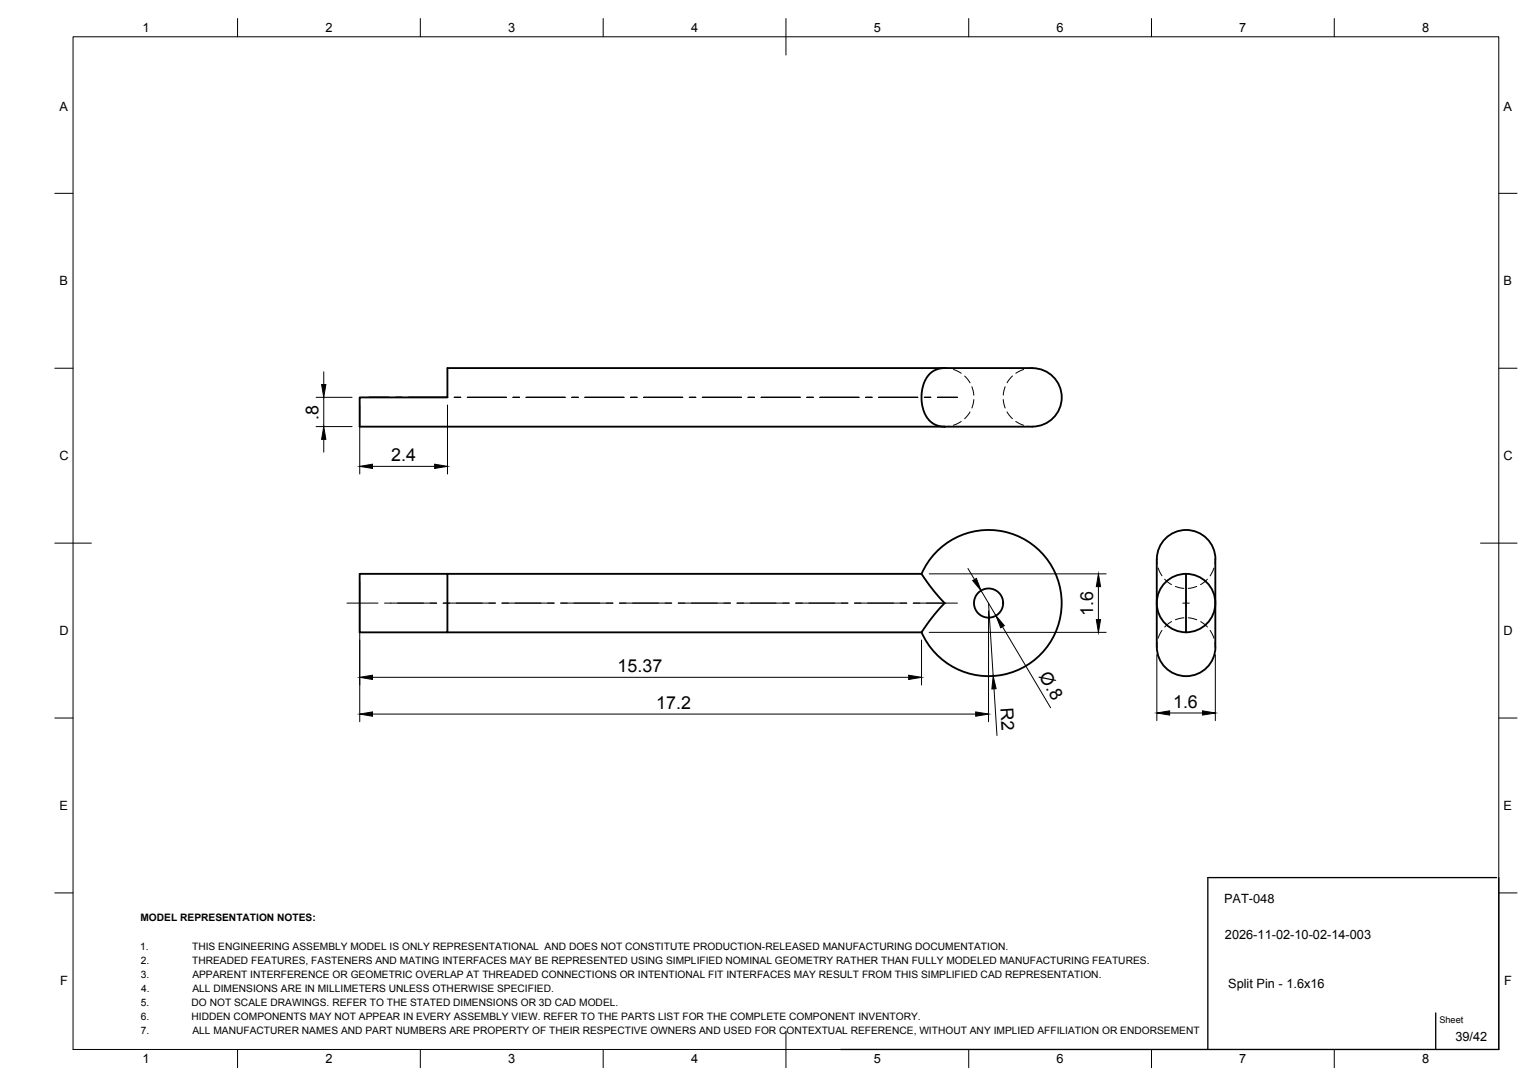
ISO-10303-21;
HEADER;
/* Generated by software containing ST-Developer
 * from STEP Tools, Inc. (www.steptools.com) 
 */

FILE_DESCRIPTION(
/* description */ ('Guided pneumatic stop gate'),
/* implementation_level */ '2;1');

FILE_NAME(
/* name */ 'Split Pin - 1.6x16.step',
/* time_stamp */ '2026-10-27T21:43:45-07:00',
/* author */ (''),
/* organization */ (''),
/* preprocessor_version */ 'ST-DEVELOPER v20.2',
/* originating_system */ 'Autodesk Translation Framework v15.17.0.0',
/* authorisation */ '');

FILE_SCHEMA (('AUTOMOTIVE_DESIGN { 1 0 10303 214 3 1 1 }'));
ENDSEC;

DATA;
#10=MECHANICAL_DESIGN_GEOMETRIC_PRESENTATION_REPRESENTATION('',(#571),#14392);
#17=B_SPLINE_CURVE_WITH_KNOTS('',3,(#14014,#14015,#14016,#14017,#14018,
#14019,#14020,#14021,#14022,#14023,#14024,#14025,#14026,#14027,#14028,#14029,
#14030,#14031,#14032,#14033,#14034,#14035,#14036,#14037,#14038,#14039),
 .UNSPECIFIED.,.F.,.F.,(4,2,2,2,2,2,2,2,2,2,2,2,4),(-0.00054581412719389,
0.,0.0281583564005144,0.0618496465371181,0.0905865724114538,0.120694112793616,
0.144966158459363,0.16923820412511,0.199345744507272,0.228082670381608,
0.261773960518212,0.289932316918681,0.290478131045882),.UNSPECIFIED.);
#18=B_SPLINE_CURVE_WITH_KNOTS('',3,(#14040,#14041,#14042,#14043,#14044,
#14045,#14046,#14047,#14048,#14049,#14050,#14051,#14052,#14053,#14054,#14055,
#14056,#14057,#14058,#14059,#14060,#14061,#14062,#14063,#14064,#14065),
 .UNSPECIFIED.,.F.,.F.,(4,2,2,2,2,2,2,2,2,2,2,2,4),(-0.000545814127196571,
0.,0.0281583564006391,0.0618496465374156,0.0905865724118984,0.120694112794215,
0.144966158460086,0.169238204125958,0.199345744508275,0.228082670382758,
0.261773960519534,0.289932316920171,0.29047813104737),.UNSPECIFIED.);
#46=TOROIDAL_SURFACE('',#9285,0.12,0.08);
#487=SHAPE_REPRESENTATION_RELATIONSHIP('SRR','None',#14624,#529);
#529=ADVANCED_BREP_SHAPE_REPRESENTATION('',(#609),#14386);
#571=STYLED_ITEM('',(#14891),#609);
#609=MANIFOLD_SOLID_BREP('Body1',#7915);
#811=FACE_BOUND('',#2221,.T.);
#1088=PLANE('',#9288);
#1089=PLANE('',#9290);
#1090=PLANE('',#9294);
#1549=FACE_OUTER_BOUND('',#2220,.T.);
#1550=FACE_OUTER_BOUND('',#2222,.T.);
#1551=FACE_OUTER_BOUND('',#2223,.T.);
#1552=FACE_OUTER_BOUND('',#2224,.T.);
#1553=FACE_OUTER_BOUND('',#2225,.T.);
#2220=EDGE_LOOP('',(#7060,#7061,#7062,#7063));
#2221=EDGE_LOOP('',(#7064,#7065));
#2222=EDGE_LOOP('',(#7066,#7067));
#2223=EDGE_LOOP('',(#7068,#7069,#7070,#7071));
#2224=EDGE_LOOP('',(#7072,#7073,#7074,#7075,#7076,#7077,#7078,#7079,#7080));
#2225=EDGE_LOOP('',(#7081,#7082,#7083));
#2776=LINE('',#14070,#3321);
#2777=LINE('',#14073,#3322);
#2778=LINE('',#14075,#3323);
#2779=LINE('',#14076,#3324);
#2780=LINE('',#14080,#3325);
#3321=VECTOR('',#11691,1.);
#3322=VECTOR('',#11694,1.);
#3323=VECTOR('',#11695,1.);
#3324=VECTOR('',#11696,1.);
#3325=VECTOR('',#11701,0.08);
#3710=CIRCLE('',#9286,0.08);
#3711=CIRCLE('',#9287,0.04);
#3712=CIRCLE('',#9289,0.08);
#3713=CIRCLE('',#9292,0.08);
#3714=CIRCLE('',#9293,0.08);
#4298=VERTEX_POINT('',#14009);
#4299=VERTEX_POINT('',#14012);
#4300=VERTEX_POINT('',#14013);
#4301=VERTEX_POINT('',#14067);
#4302=VERTEX_POINT('',#14068);
#4303=VERTEX_POINT('',#14072);
#4304=VERTEX_POINT('',#14074);
#4305=VERTEX_POINT('',#14078);
#5228=EDGE_CURVE('',#4298,#4298,#3710,.T.);
#5229=EDGE_CURVE('',#4298,#4298,#3711,.T.);
#5230=EDGE_CURVE('',#4299,#4300,#17,.T.);
#5231=EDGE_CURVE('',#4300,#4299,#18,.T.);
#5232=EDGE_CURVE('',#4301,#4302,#3712,.T.);
#5233=EDGE_CURVE('',#4301,#4302,#2776,.T.);
#5234=EDGE_CURVE('',#4302,#4303,#2777,.T.);
#5235=EDGE_CURVE('',#4304,#4303,#2778,.T.);
#5236=EDGE_CURVE('',#4301,#4304,#2779,.T.);
#5237=EDGE_CURVE('',#4305,#4304,#3713,.T.);
#5238=EDGE_CURVE('',#4305,#4300,#2780,.T.);
#5239=EDGE_CURVE('',#4303,#4305,#3714,.T.);
#7060=ORIENTED_EDGE('',*,*,#5228,.F.);
#7061=ORIENTED_EDGE('',*,*,#5229,.T.);
#7062=ORIENTED_EDGE('',*,*,#5228,.T.);
#7063=ORIENTED_EDGE('',*,*,#5229,.F.);
#7064=ORIENTED_EDGE('',*,*,#5230,.F.);
#7065=ORIENTED_EDGE('',*,*,#5231,.F.);
#7066=ORIENTED_EDGE('',*,*,#5232,.T.);
#7067=ORIENTED_EDGE('',*,*,#5233,.F.);
#7068=ORIENTED_EDGE('',*,*,#5233,.T.);
#7069=ORIENTED_EDGE('',*,*,#5234,.T.);
#7070=ORIENTED_EDGE('',*,*,#5235,.F.);
#7071=ORIENTED_EDGE('',*,*,#5236,.F.);
#7072=ORIENTED_EDGE('',*,*,#5232,.F.);
#7073=ORIENTED_EDGE('',*,*,#5236,.T.);
#7074=ORIENTED_EDGE('',*,*,#5237,.F.);
#7075=ORIENTED_EDGE('',*,*,#5238,.T.);
#7076=ORIENTED_EDGE('',*,*,#5231,.T.);
#7077=ORIENTED_EDGE('',*,*,#5230,.T.);
#7078=ORIENTED_EDGE('',*,*,#5238,.F.);
#7079=ORIENTED_EDGE('',*,*,#5239,.F.);
#7080=ORIENTED_EDGE('',*,*,#5234,.F.);
#7081=ORIENTED_EDGE('',*,*,#5239,.T.);
#7082=ORIENTED_EDGE('',*,*,#5237,.T.);
#7083=ORIENTED_EDGE('',*,*,#5235,.T.);
#7389=CYLINDRICAL_SURFACE('',#9291,0.08);
#7831=ADVANCED_FACE('',(#1549,#811),#46,.T.);
#7832=ADVANCED_FACE('',(#1550),#1088,.F.);
#7833=ADVANCED_FACE('',(#1551),#1089,.T.);
#7834=ADVANCED_FACE('',(#1552),#7389,.T.);
#7835=ADVANCED_FACE('',(#1553),#1090,.F.);
#7915=CLOSED_SHELL('',(#7831,#7832,#7833,#7834,#7835));
#9284=AXIS2_PLACEMENT_3D('',#14007,#11679,#11680);
#9285=AXIS2_PLACEMENT_3D('',#14008,#11681,#11682);
#9286=AXIS2_PLACEMENT_3D('',#14010,#11683,#11684);
#9287=AXIS2_PLACEMENT_3D('',#14011,#11685,#11686);
#9288=AXIS2_PLACEMENT_3D('',#14066,#11687,#11688);
#9289=AXIS2_PLACEMENT_3D('',#14069,#11689,#11690);
#9290=AXIS2_PLACEMENT_3D('',#14071,#11692,#11693);
#9291=AXIS2_PLACEMENT_3D('',#14077,#11697,#11698);
#9292=AXIS2_PLACEMENT_3D('',#14079,#11699,#11700);
#9293=AXIS2_PLACEMENT_3D('',#14081,#11702,#11703);
#9294=AXIS2_PLACEMENT_3D('',#14082,#11704,#11705);
#11679=DIRECTION('axis',(0.,0.,1.));
#11680=DIRECTION('refdir',(1.,0.,0.));
#11681=DIRECTION('center_axis',(-1.,0.,0.));
#11682=DIRECTION('ref_axis',(0.,0.,1.));
#11683=DIRECTION('center_axis',(0.,-1.,1.38777878078145E-16));
#11684=DIRECTION('ref_axis',(0.,-1.38777878078145E-16,-1.));
#11685=DIRECTION('center_axis',(1.,0.,0.));
#11686=DIRECTION('ref_axis',(0.,0.,1.));
#11687=DIRECTION('center_axis',(0.,1.,0.));
#11688=DIRECTION('ref_axis',(1.,0.,0.));
#11689=DIRECTION('center_axis',(0.,-1.,0.));
#11690=DIRECTION('ref_axis',(1.,0.,0.));
#11691=DIRECTION('',(0.,0.,1.));
#11692=DIRECTION('center_axis',(1.,0.,0.));
#11693=DIRECTION('ref_axis',(0.,0.,1.));
#11694=DIRECTION('',(0.,-1.,0.));
#11695=DIRECTION('',(0.,0.,1.));
#11696=DIRECTION('',(0.,-1.,0.));
#11697=DIRECTION('center_axis',(0.,-1.,0.));
#11698=DIRECTION('ref_axis',(1.,0.,0.));
#11699=DIRECTION('center_axis',(0.,-1.,0.));
#11700=DIRECTION('ref_axis',(1.,0.,0.));
#11701=DIRECTION('',(0.,1.,0.));
#11702=DIRECTION('center_axis',(0.,-1.,0.));
#11703=DIRECTION('ref_axis',(1.,0.,0.));
#11704=DIRECTION('center_axis',(0.,1.,0.));
#11705=DIRECTION('ref_axis',(1.,0.,0.));
#14007=CARTESIAN_POINT('',(0.,0.,0.));
#14008=CARTESIAN_POINT('Origin',(0.,0.12,0.));
#14009=CARTESIAN_POINT('',(-9.79717439317883E-18,0.12,-0.04));
#14010=CARTESIAN_POINT('Origin',(0.,0.12,-0.12));
#14011=CARTESIAN_POINT('Origin',(9.79717439317883E-18,0.12,0.));
#14012=CARTESIAN_POINT('',(0.08,-4.89858719658941E-18,7.34788079488412E-18));
#14013=CARTESIAN_POINT('',(-0.08,-4.89858719658941E-18,7.34788079488412E-18));
#14014=CARTESIAN_POINT('Ctrl Pts',(0.08,-4.89858719658941E-18,7.34788079488412E-18));
#14015=CARTESIAN_POINT('Ctrl Pts',(0.08,-0.00012864962353541,0.000128649623535413));
#14016=CARTESIAN_POINT('Ctrl Pts',(0.0799996896739287,-0.00025719571182076,
0.000257402596003253));
#14017=CARTESIAN_POINT('Ctrl Pts',(0.0799669711262291,-0.00701193164572964,
0.00703384588894362));
#14018=CARTESIAN_POINT('Ctrl Pts',(0.0791054994909294,-0.0133457972655825,
0.0139383126556792));
#14019=CARTESIAN_POINT('Ctrl Pts',(0.0749700088488058,-0.0265076530862524,
0.0292212026164895));
#14020=CARTESIAN_POINT('Ctrl Pts',(0.0712702072865517,-0.0331317062461458,
0.0375603420117568));
#14021=CARTESIAN_POINT('Ctrl Pts',(0.0612858949407667,-0.0440683985740427,
0.0520545604187517));
#14022=CARTESIAN_POINT('Ctrl Pts',(0.0555090276731744,-0.0485199197794574,
0.0582717815295611));
#14023=CARTESIAN_POINT('Ctrl Pts',(0.0412398082144208,-0.0561090538733877,
0.0691638397919718));
#14024=CARTESIAN_POINT('Ctrl Pts',(0.0327878980890048,-0.059089642483296,
0.0736229049587921));
#14025=CARTESIAN_POINT('Ctrl Pts',(0.0159233027310102,-0.0625179833270725,
0.0787936360751706));
#14026=CARTESIAN_POINT('Ctrl Pts',(0.00801661414593076,-0.0633030277982336,
0.08));
#14027=CARTESIAN_POINT('Ctrl Pts',(-0.00801661414593074,-0.0633030277982336,
0.08));
#14028=CARTESIAN_POINT('Ctrl Pts',(-0.0159233027310102,-0.0625179833270726,
0.0787936360751706));
#14029=CARTESIAN_POINT('Ctrl Pts',(-0.0327878980890049,-0.059089642483296,
0.0736229049587921));
#14030=CARTESIAN_POINT('Ctrl Pts',(-0.0412398082144209,-0.0561090538733877,
0.0691638397919717));
#14031=CARTESIAN_POINT('Ctrl Pts',(-0.0555090276731744,-0.0485199197794574,
0.0582717815295611));
#14032=CARTESIAN_POINT('Ctrl Pts',(-0.0612858949407667,-0.0440683985740427,
0.0520545604187517));
#14033=CARTESIAN_POINT('Ctrl Pts',(-0.0712702072865517,-0.0331317062461458,
0.0375603420117568));
#14034=CARTESIAN_POINT('Ctrl Pts',(-0.0749700088488058,-0.0265076530862524,
0.0292212026164895));
#14035=CARTESIAN_POINT('Ctrl Pts',(-0.0791054994909264,-0.0133457972655921,
0.0139383126556903));
#14036=CARTESIAN_POINT('Ctrl Pts',(-0.0799669711262287,-0.00701193164579759,
0.0070338458890125));
#14037=CARTESIAN_POINT('Ctrl Pts',(-0.0799996896739287,-0.000257195711817665,
0.000257402596000083));
#14038=CARTESIAN_POINT('Ctrl Pts',(-0.08,-0.000128649623538514,0.000128649623538516));
#14039=CARTESIAN_POINT('Ctrl Pts',(-0.08,-4.89858719658941E-18,7.34788079488412E-18));
#14040=CARTESIAN_POINT('Ctrl Pts',(-0.08,-4.89858719658941E-18,7.34788079488412E-18));
#14041=CARTESIAN_POINT('Ctrl Pts',(-0.08,-0.000128649623536042,-0.00012864962353603));
#14042=CARTESIAN_POINT('Ctrl Pts',(-0.0799996896739287,-0.000257195711820127,
-0.000257402596002604));
#14043=CARTESIAN_POINT('Ctrl Pts',(-0.0799669711262289,-0.0070119316457589,
-0.00703384588897312));
#14044=CARTESIAN_POINT('Ctrl Pts',(-0.0791054994909281,-0.0133457972655867,
-0.0139383126556841));
#14045=CARTESIAN_POINT('Ctrl Pts',(-0.0749700088488058,-0.0265076530862525,
-0.0292212026164896));
#14046=CARTESIAN_POINT('Ctrl Pts',(-0.0712702072865516,-0.0331317062461459,
-0.0375603420117568));
#14047=CARTESIAN_POINT('Ctrl Pts',(-0.0612858949407667,-0.0440683985740427,
-0.0520545604187517));
#14048=CARTESIAN_POINT('Ctrl Pts',(-0.0555090276731744,-0.0485199197794574,
-0.0582717815295611));
#14049=CARTESIAN_POINT('Ctrl Pts',(-0.0412398082144209,-0.0561090538733877,
-0.0691638397919717));
#14050=CARTESIAN_POINT('Ctrl Pts',(-0.0327878980890049,-0.059089642483296,
-0.0736229049587921));
#14051=CARTESIAN_POINT('Ctrl Pts',(-0.0159233027310101,-0.0625179833270725,
-0.0787936360751706));
#14052=CARTESIAN_POINT('Ctrl Pts',(-0.00801661414593069,-0.0633030277982336,
-0.08));
#14053=CARTESIAN_POINT('Ctrl Pts',(0.0080166141459307,-0.0633030277982336,
-0.08));
#14054=CARTESIAN_POINT('Ctrl Pts',(0.0159233027310101,-0.0625179833270725,
-0.0787936360751706));
#14055=CARTESIAN_POINT('Ctrl Pts',(0.0327878980890049,-0.0590896424832959,
-0.0736229049587921));
#14056=CARTESIAN_POINT('Ctrl Pts',(0.0412398082144209,-0.0561090538733877,
-0.0691638397919717));
#14057=CARTESIAN_POINT('Ctrl Pts',(0.0555090276731744,-0.0485199197794574,
-0.0582717815295611));
#14058=CARTESIAN_POINT('Ctrl Pts',(0.0612858949407666,-0.0440683985740428,
-0.0520545604187518));
#14059=CARTESIAN_POINT('Ctrl Pts',(0.0712702072865517,-0.0331317062461458,
-0.0375603420117568));
#14060=CARTESIAN_POINT('Ctrl Pts',(0.0749700088488058,-0.0265076530862524,
-0.0292212026164895));
#14061=CARTESIAN_POINT('Ctrl Pts',(0.079105499490928,-0.013345797265587,
-0.0139383126556845));
#14062=CARTESIAN_POINT('Ctrl Pts',(0.0799669711262289,-0.00701193164576148,
-0.00703384588897579));
#14063=CARTESIAN_POINT('Ctrl Pts',(0.0799996896739287,-0.000257195711819584,
-0.000257402596002039));
#14064=CARTESIAN_POINT('Ctrl Pts',(0.08,-0.000128649623536605,-0.000128649623536593));
#14065=CARTESIAN_POINT('Ctrl Pts',(0.08,-4.89858719658941E-18,7.34788079488412E-18));
#14066=CARTESIAN_POINT('Origin',(0.04,-1.36,0.));
#14067=CARTESIAN_POINT('',(0.,-1.36,-0.08));
#14068=CARTESIAN_POINT('',(0.,-1.36,0.08));
#14069=CARTESIAN_POINT('Origin',(0.,-1.36,0.));
#14070=CARTESIAN_POINT('',(0.,-1.36,-0.04));
#14071=CARTESIAN_POINT('Origin',(0.,0.,-0.08));
#14072=CARTESIAN_POINT('',(0.,-1.6,0.08));
#14073=CARTESIAN_POINT('',(0.,0.,0.08));
#14074=CARTESIAN_POINT('',(0.,-1.6,-0.08));
#14075=CARTESIAN_POINT('',(0.,-1.6,-0.09));
#14076=CARTESIAN_POINT('',(0.,0.,-0.08));
#14077=CARTESIAN_POINT('Origin',(0.,0.,0.));
#14078=CARTESIAN_POINT('',(-0.08,-1.6,-9.79717439317883E-18));
#14079=CARTESIAN_POINT('Origin',(0.,-1.6,0.));
#14080=CARTESIAN_POINT('',(-0.08,0.,-9.79717439317883E-18));
#14081=CARTESIAN_POINT('Origin',(0.,-1.6,0.));
#14082=CARTESIAN_POINT('Origin',(-0.04,-1.6,0.));
#14338=UNCERTAINTY_MEASURE_WITH_UNIT(LENGTH_MEASURE(0.001),#14393,
'DISTANCE_ACCURACY_VALUE',
'Maximum model space distance between geometric entities at asserted c
onnectivities');
#14344=UNCERTAINTY_MEASURE_WITH_UNIT(LENGTH_MEASURE(0.001),#14393,
'DISTANCE_ACCURACY_VALUE',
'Maximum model space distance between geometric entities at asserted c
onnectivities');
#14386=(
GEOMETRIC_REPRESENTATION_CONTEXT(3)
GLOBAL_UNCERTAINTY_ASSIGNED_CONTEXT((#14338))
GLOBAL_UNIT_ASSIGNED_CONTEXT((#14393,#14395,#14396))
REPRESENTATION_CONTEXT('','3D')
);
#14392=(
GEOMETRIC_REPRESENTATION_CONTEXT(3)
GLOBAL_UNCERTAINTY_ASSIGNED_CONTEXT((#14344))
GLOBAL_UNIT_ASSIGNED_CONTEXT((#14393,#14395,#14396))
REPRESENTATION_CONTEXT('','3D')
);
#14393=(
LENGTH_UNIT()
NAMED_UNIT(*)
SI_UNIT(.CENTI.,.METRE.)
);
#14395=(
NAMED_UNIT(*)
PLANE_ANGLE_UNIT()
SI_UNIT($,.RADIAN.)
);
#14396=(
NAMED_UNIT(*)
SI_UNIT($,.STERADIAN.)
SOLID_ANGLE_UNIT()
);
#14438=SHAPE_DEFINITION_REPRESENTATION(#14557,#14624);
#14557=PRODUCT_DEFINITION_SHAPE('',$,#14672);
#14624=SHAPE_REPRESENTATION('',(#9284),#14386);
#14630=PRODUCT_DEFINITION_CONTEXT('part definition',#14773,'design');
#14672=PRODUCT_DEFINITION('Split Pin - 1.6x16','Split Pin - 1.6x16',#14719,
#14630);
#14719=PRODUCT_DEFINITION_FORMATION('',$,#14816);
#14773=APPLICATION_CONTEXT(
'Core Data for Automotive Mechanical Design Process');
#14774=PRODUCT_CONTEXT('part definition',#14773,'mechanical');
#14816=PRODUCT('Split Pin - 1.6x16','Split Pin - 1.6x16',
'Split Pin - 1.6x16',(#14774));
#14885=COLOUR_RGB('Grey',0.48,0.52,0.57);
#14886=FILL_AREA_STYLE_COLOUR('',#14885);
#14887=FILL_AREA_STYLE('',(#14886));
#14888=SURFACE_STYLE_FILL_AREA(#14887);
#14889=SURFACE_SIDE_STYLE('',(#14888));
#14890=SURFACE_STYLE_USAGE(.BOTH.,#14889);
#14891=PRESENTATION_STYLE_ASSIGNMENT((#14890));
ENDSEC;
END-ISO-10303-21;
